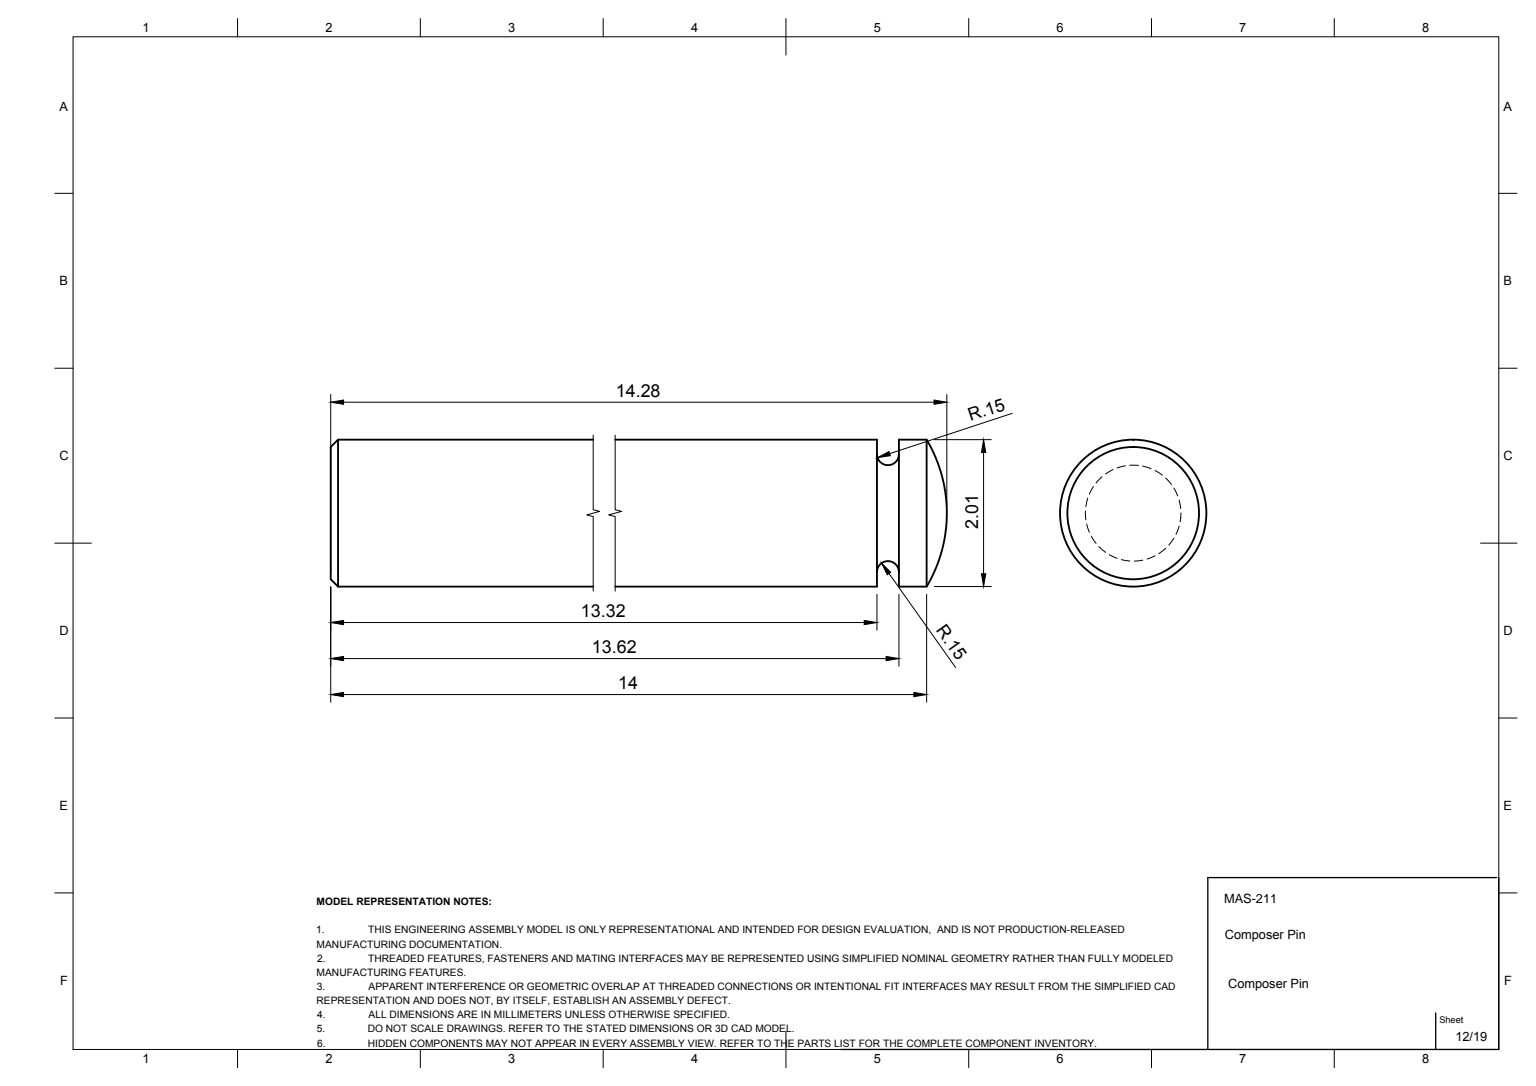
ISO-10303-21;
HEADER;
FILE_DESCRIPTION(
 (''),
 '2;1');
FILE_NAME ( 'Composer Pin.step', '2026-10-05T20:07:59+06:00', ( '' ), ( '' ), 'STEP AP214', 'Unspecified', '' );
FILE_SCHEMA (('AUTOMOTIVE_DESIGN { 1 0 10303 214 3 1 1 }'));
ENDSEC;
DATA;
#10=MECHANICAL_DESIGN_GEOMETRIC_PRESENTATION_REPRESENTATION('',(#329),#196741);
#17=(
BOUNDED_CURVE()
B_SPLINE_CURVE(2,(#114139,#114140,#114141,#114142,#114143,#114144,#114145,
#114146,#114147),.UNSPECIFIED.,.F.,.F.)
B_SPLINE_CURVE_WITH_KNOTS((3,2,2,2,3),(1.42918797785348,1.62618617063892,
1.86180561965816,2.09742506867739,2.29442326146283),.UNSPECIFIED.)
CURVE()
GEOMETRIC_REPRESENTATION_ITEM()
RATIONAL_B_SPLINE_CURVE((1.,1.,1.,0.707106781186548,1.,0.707106781186548,
1.,1.,1.))
REPRESENTATION_ITEM('')
) ;
#33=(
BOUNDED_SURFACE()
B_SPLINE_SURFACE(2,2,((#114004,#114005,#114006,#114007,#114008,#114009,
#114010,#114011,#114012),(#114013,#114014,#114015,#114016,#114017,#114018,
#114019,#114020,#114021),(#114022,#114023,#114024,#114025,#114026,#114027,
#114028,#114029,#114030)),.UNSPECIFIED.,.F.,.T.,.F.)
B_SPLINE_SURFACE_WITH_KNOTS((3,3),(3,2,2,2,3),(0.,1.05013832301181),(0.,
1.5707963267949,3.1415926535898,4.71238898038469,6.28318530717959),
 .UNSPECIFIED.)
GEOMETRIC_REPRESENTATION_ITEM()
RATIONAL_B_SPLINE_SURFACE(((1.,0.707106781186548,1.,0.707106781186548,1.,
0.707106781186548,1.,0.707106781186548,1.),(0.963886720506905,0.681570836366095,
0.963886720506905,0.681570836366095,0.963886720506905,0.681570836366095,
0.963886720506905,0.681570836366095,0.963886720506905),(1.,0.707106781186548,
1.,0.707106781186548,1.,0.707106781186548,1.,0.707106781186548,1.)))
REPRESENTATION_ITEM('')
SURFACE()
) ;
#34=(
BOUNDED_SURFACE()
B_SPLINE_SURFACE(2,1,((#114035,#114036),(#114037,#114038),(#114039,#114040),
(#114041,#114042),(#114043,#114044),(#114045,#114046),(#114047,#114048),
(#114049,#114050),(#114051,#114052)),.UNSPECIFIED.,.T.,.F.,.F.)
B_SPLINE_SURFACE_WITH_KNOTS((3,2,2,2,3),(2,2),(0.,1.5707963267949,3.1415926535898,
4.71238898038469,6.28318530717959),(0.,0.0454859585810009),
 .UNSPECIFIED.)
GEOMETRIC_REPRESENTATION_ITEM()
RATIONAL_B_SPLINE_SURFACE(((1.,1.),(0.707106781186548,0.707106781186548),
(1.,1.),(0.707106781186548,0.707106781186548),(1.,1.),(0.707106781186548,
0.707106781186548),(1.,1.),(0.707106781186548,0.707106781186548),(1.,1.)))
REPRESENTATION_ITEM('')
SURFACE()
) ;
#35=(
BOUNDED_SURFACE()
B_SPLINE_SURFACE(2,2,((#114056,#114057,#114058,#114059,#114060,#114061,
#114062,#114063,#114064),(#114065,#114066,#114067,#114068,#114069,#114070,
#114071,#114072,#114073),(#114074,#114075,#114076,#114077,#114078,#114079,
#114080,#114081,#114082),(#114083,#114084,#114085,#114086,#114087,#114088,
#114089,#114090,#114091),(#114092,#114093,#114094,#114095,#114096,#114097,
#114098,#114099,#114100),(#114101,#114102,#114103,#114104,#114105,#114106,
#114107,#114108,#114109),(#114110,#114111,#114112,#114113,#114114,#114115,
#114116,#114117,#114118),(#114119,#114120,#114121,#114122,#114123,#114124,
#114125,#114126,#114127),(#114128,#114129,#114130,#114131,#114132,#114133,
#114134,#114135,#114136)),.UNSPECIFIED.,.F.,.T.,.F.)
B_SPLINE_SURFACE_WITH_KNOTS((3,2,2,2,3),(3,2,2,2,3),(1.42918797785348,1.62618617063892,
1.86180561965816,2.09742506867739,2.29442326146283),(0.,1.5707963267949,
3.1415926535898,4.71238898038469,6.28318530717959),.UNSPECIFIED.)
GEOMETRIC_REPRESENTATION_ITEM()
RATIONAL_B_SPLINE_SURFACE(((1.,0.707106781186548,1.,0.707106781186548,1.,
0.707106781186548,1.,0.707106781186548,1.),(1.,0.707106781186548,1.,0.707106781186548,
1.,0.707106781186548,1.,0.707106781186548,1.),(1.,0.707106781186548,1.,
0.707106781186548,1.,0.707106781186548,1.,0.707106781186548,1.),(0.707106781186548,
0.5,0.707106781186548,0.5,0.707106781186548,0.5,0.707106781186548,0.5,0.707106781186548),
(1.,0.707106781186548,1.,0.707106781186548,1.,0.707106781186548,1.,0.707106781186548,
1.),(0.707106781186548,0.5,0.707106781186548,0.5,0.707106781186548,0.5,
0.707106781186548,0.5,0.707106781186548),(1.,0.707106781186548,1.,0.707106781186548,
1.,0.707106781186548,1.,0.707106781186548,1.),(1.,0.707106781186548,1.,
0.707106781186548,1.,0.707106781186548,1.,0.707106781186548,1.),(1.,0.707106781186548,
1.,0.707106781186548,1.,0.707106781186548,1.,0.707106781186548,1.)))
REPRESENTATION_ITEM('')
SURFACE()
) ;
#36=(
BOUNDED_SURFACE()
B_SPLINE_SURFACE(2,1,((#114148,#114149),(#114150,#114151),(#114152,#114153),
(#114154,#114155),(#114156,#114157),(#114158,#114159),(#114160,#114161),
(#114162,#114163),(#114164,#114165)),.UNSPECIFIED.,.T.,.F.,.F.)
B_SPLINE_SURFACE_WITH_KNOTS((3,2,2,2,3),(2,2),(0.,1.5707963267949,3.1415926535898,
4.71238898038469,6.28318530717959),(0.,1.586514041419),.UNSPECIFIED.)
GEOMETRIC_REPRESENTATION_ITEM()
RATIONAL_B_SPLINE_SURFACE(((1.,1.),(0.707106781186548,0.707106781186548),
(1.,1.),(0.707106781186548,0.707106781186548),(1.,1.),(0.707106781186548,
0.707106781186548),(1.,1.),(0.707106781186548,0.707106781186548),(1.,1.)))
REPRESENTATION_ITEM('')
SURFACE()
) ;
#37=(
BOUNDED_SURFACE()
B_SPLINE_SURFACE(1,2,((#114169,#114170,#114171,#114172,#114173,#114174,
#114175,#114176,#114177),(#114178,#114179,#114180,#114181,#114182,#114183,
#114184,#114185,#114186)),.UNSPECIFIED.,.F.,.T.,.F.)
B_SPLINE_SURFACE_WITH_KNOTS((2,2),(3,2,2,2,3),(15.5153736066212,15.6567949628585),
(0.,1.5707963267949,3.1415926535898,4.71238898038469,6.28318530717959),
 .UNSPECIFIED.)
GEOMETRIC_REPRESENTATION_ITEM()
RATIONAL_B_SPLINE_SURFACE(((1.,0.707106781186548,1.,0.707106781186548,1.,
0.707106781186548,1.,0.707106781186548,1.),(1.,0.707106781186548,1.,0.707106781186548,
1.,0.707106781186548,1.,0.707106781186548,1.)))
REPRESENTATION_ITEM('')
SURFACE()
) ;
#139=ELLIPSE('',#8975,0.90392506178254,0.899999999999994) ;
#140=ELLIPSE('',#8976,1.00436117975839,0.999999999999988) ;
#141=ELLIPSE('',#8978,1.00436117975839,0.999999999999988) ;
#142=ELLIPSE('',#8979,1.00436117975839,0.999999999999988) ;
#143=ELLIPSE('',#8980,1.00436117975839,0.999999999999998) ;
#329=STYLED_ITEM('',(#196765),#348) ;
#348=MANIFOLD_SOLID_BREP('Composer Pin',#8725) ;
#398=PLANE('',#8974) ;
#707=CIRCLE('',#8977,1.94783572104092) ;
#1030=FACE_OUTER_BOUND('',#1539,.T.) ;
#1031=FACE_OUTER_BOUND('',#1540,.T.) ;
#1032=FACE_OUTER_BOUND('',#1541,.T.) ;
#1033=FACE_OUTER_BOUND('',#1542,.T.) ;
#1034=FACE_OUTER_BOUND('',#1543,.T.) ;
#1035=FACE_OUTER_BOUND('',#1544,.T.) ;
#1539=EDGE_LOOP('',(#6448,#6449,#6450)) ;
#1540=EDGE_LOOP('',(#6451,#6452,#6453)) ;
#1541=EDGE_LOOP('',(#6454,#6455,#6456,#6457)) ;
#1542=EDGE_LOOP('',(#6458,#6459,#6460,#6461)) ;
#1543=EDGE_LOOP('',(#6462,#6463,#6464,#6465)) ;
#1544=EDGE_LOOP('',(#6466,#6467,#6468,#6469)) ;
#2034=LINE('',#114002,#2737) ;
#2035=LINE('',#114055,#2738) ;
#2036=LINE('',#114168,#2739) ;
#2037=LINE('',#114187,#2740) ;
#2737=VECTOR('',#10084,10.) ;
#2738=VECTOR('',#10093,10.) ;
#2739=VECTOR('',#10098,10.) ;
#2740=VECTOR('',#10099,10.) ;
#3736=VERTEX_POINT('',#114000) ;
#3737=VERTEX_POINT('',#114001) ;
#3738=VERTEX_POINT('',#114031) ;
#3739=VERTEX_POINT('',#114033) ;
#3740=VERTEX_POINT('',#114053) ;
#3741=VERTEX_POINT('',#114137) ;
#3742=VERTEX_POINT('',#114166) ;
#4732=EDGE_CURVE('',#3736,#3737,#2034,.T.) ;
#4733=EDGE_CURVE('',#3736,#3736,#139,.T.) ;
#4734=EDGE_CURVE('',#3738,#3738,#140,.T.) ;
#4735=EDGE_CURVE('',#3739,#3738,#707,.T.) ;
#4736=EDGE_CURVE('',#3740,#3740,#141,.T.) ;
#4737=EDGE_CURVE('',#3738,#3740,#2035,.T.) ;
#4738=EDGE_CURVE('',#3741,#3741,#142,.T.) ;
#4739=EDGE_CURVE('',#3740,#3741,#17,.T.) ;
#4740=EDGE_CURVE('',#3742,#3742,#143,.T.) ;
#4741=EDGE_CURVE('',#3741,#3742,#2036,.T.) ;
#4742=EDGE_CURVE('',#3742,#3736,#2037,.T.) ;
#6448=ORIENTED_EDGE('',*,*,#4732,.T.) ;
#6449=ORIENTED_EDGE('',*,*,#4732,.F.) ;
#6450=ORIENTED_EDGE('',*,*,#4733,.F.) ;
#6451=ORIENTED_EDGE('',*,*,#4734,.T.) ;
#6452=ORIENTED_EDGE('',*,*,#4735,.F.) ;
#6453=ORIENTED_EDGE('',*,*,#4735,.T.) ;
#6454=ORIENTED_EDGE('',*,*,#4736,.T.) ;
#6455=ORIENTED_EDGE('',*,*,#4737,.F.) ;
#6456=ORIENTED_EDGE('',*,*,#4734,.F.) ;
#6457=ORIENTED_EDGE('',*,*,#4737,.T.) ;
#6458=ORIENTED_EDGE('',*,*,#4738,.T.) ;
#6459=ORIENTED_EDGE('',*,*,#4739,.F.) ;
#6460=ORIENTED_EDGE('',*,*,#4736,.F.) ;
#6461=ORIENTED_EDGE('',*,*,#4739,.T.) ;
#6462=ORIENTED_EDGE('',*,*,#4740,.T.) ;
#6463=ORIENTED_EDGE('',*,*,#4741,.F.) ;
#6464=ORIENTED_EDGE('',*,*,#4738,.F.) ;
#6465=ORIENTED_EDGE('',*,*,#4741,.T.) ;
#6466=ORIENTED_EDGE('',*,*,#4733,.T.) ;
#6467=ORIENTED_EDGE('',*,*,#4742,.F.) ;
#6468=ORIENTED_EDGE('',*,*,#4740,.F.) ;
#6469=ORIENTED_EDGE('',*,*,#4742,.T.) ;
#8413=ADVANCED_FACE('',(#1030),#398,.T.) ;
#8414=ADVANCED_FACE('',(#1031),#33,.T.) ;
#8415=ADVANCED_FACE('',(#1032),#34,.F.) ;
#8416=ADVANCED_FACE('',(#1033),#35,.T.) ;
#8417=ADVANCED_FACE('',(#1034),#36,.F.) ;
#8418=ADVANCED_FACE('',(#1035),#37,.T.) ;
#8725=CLOSED_SHELL('',(#8413,#8414,#8415,#8416,#8417,#8418)) ;
#8974=AXIS2_PLACEMENT_3D('',#113999,#10082,#10083) ;
#8975=AXIS2_PLACEMENT_3D('',#114003,#10085,#10086) ;
#8976=AXIS2_PLACEMENT_3D('',#114032,#10087,#10088) ;
#8977=AXIS2_PLACEMENT_3D('',#114034,#10089,#10090) ;
#8978=AXIS2_PLACEMENT_3D('',#114054,#10091,#10092) ;
#8979=AXIS2_PLACEMENT_3D('',#114138,#10094,#10095) ;
#8980=AXIS2_PLACEMENT_3D('',#114167,#10096,#10097) ;
#10082=DIRECTION('center_axis',(-4.35747896024226E-15,-1.,5.94017881872706E-16)) ;
#10083=DIRECTION('ref_axis',(0.,-5.94017881872706E-16,-1.)) ;
#10084=DIRECTION('',(0.323867587736079,-1.97204328484321E-15,-0.946102418141933)) ;
#10085=DIRECTION('center_axis',(0.,1.,0.)) ;
#10086=DIRECTION('ref_axis',(0.946102418142542,0.,0.3238675877343)) ;
#10087=DIRECTION('center_axis',(1.67995222306785E-15,1.,-3.91636034436018E-16)) ;
#10088=DIRECTION('ref_axis',(0.946102418142689,-1.46256864286623E-15,0.323867587733871)) ;
#10089=DIRECTION('center_axis',(0.946102418141937,-3.68441630821444E-14,
0.323867587736069)) ;
#10090=DIRECTION('ref_axis',(-0.166270483818289,0.858155219939116,0.485719821195387)) ;
#10091=DIRECTION('center_axis',(1.78081198063816E-15,1.,9.26117405585395E-16)) ;
#10092=DIRECTION('ref_axis',(0.946102418142689,-1.98476993124453E-15,0.323867587733871)) ;
#10093=DIRECTION('',(-2.3431716883402E-14,-1.,4.6863433766804E-14)) ;
#10094=DIRECTION('center_axis',(1.67995222306785E-15,1.,-3.91636034436018E-16)) ;
#10095=DIRECTION('ref_axis',(0.946102418142689,-1.46256864286623E-15,0.323867587733871)) ;
#10096=DIRECTION('center_axis',(0.,1.,0.)) ;
#10097=DIRECTION('ref_axis',(0.94610241814253,0.,0.323867587734335)) ;
#10098=DIRECTION('',(-6.71796199601783E-16,-1.,1.34359239920357E-15)) ;
#10099=DIRECTION('',(0.229008967494671,-0.707106781186611,-0.668995435565098)) ;
#113999=CARTESIAN_POINT('Origin',(-34.1140302566115,0.00967047744422178,
126.985310472154)) ;
#114000=CARTESIAN_POINT('',(-34.2597706710927,0.00967047744422267,127.411056560318)) ;
#114001=CARTESIAN_POINT('',(-33.9682898421302,0.00967047744422267,126.55956438399)) ;
#114002=CARTESIAN_POINT('',(-34.2597706710927,0.00967047744422267,127.411056560318)) ;
#114003=CARTESIAN_POINT('Origin',(-33.9682898421302,0.00967047744422267,
126.55956438399)) ;
#114004=CARTESIAN_POINT('Ctrl Pts',(-33.9682898421302,14.28596080689,126.55956438399)) ;
#114005=CARTESIAN_POINT('Ctrl Pts',(-33.9682898421302,14.28596080689,126.55956438399)) ;
#114006=CARTESIAN_POINT('Ctrl Pts',(-33.9682898421302,14.28596080689,126.55956438399)) ;
#114007=CARTESIAN_POINT('Ctrl Pts',(-33.9682898421302,14.28596080689,126.55956438399)) ;
#114008=CARTESIAN_POINT('Ctrl Pts',(-33.9682898421302,14.28596080689,126.55956438399)) ;
#114009=CARTESIAN_POINT('Ctrl Pts',(-33.9682898421302,14.28596080689,126.55956438399)) ;
#114010=CARTESIAN_POINT('Ctrl Pts',(-33.9682898421302,14.28596080689,126.55956438399)) ;
#114011=CARTESIAN_POINT('Ctrl Pts',(-33.9682898421302,14.28596080689,126.55956438399)) ;
#114012=CARTESIAN_POINT('Ctrl Pts',(-33.9682898421302,14.28596080689,126.55956438399)) ;
#114013=CARTESIAN_POINT('Ctrl Pts',(-34.1425850701396,14.28596080689,127.068726593901)) ;
#114014=CARTESIAN_POINT('Ctrl Pts',(-33.631202312305,14.28596080689,127.243781954731)) ;
#114015=CARTESIAN_POINT('Ctrl Pts',(-33.4569070842956,14.28596080689,126.73461974482)) ;
#114016=CARTESIAN_POINT('Ctrl Pts',(-33.2826118562863,14.28596080689,126.225457534909)) ;
#114017=CARTESIAN_POINT('Ctrl Pts',(-33.7939946141209,14.28596080689,126.050402174079)) ;
#114018=CARTESIAN_POINT('Ctrl Pts',(-34.3053773719555,14.28596080689,125.875346813249)) ;
#114019=CARTESIAN_POINT('Ctrl Pts',(-34.4796725999648,14.28596080689,126.38450902316)) ;
#114020=CARTESIAN_POINT('Ctrl Pts',(-34.6539678279742,14.28596080689,126.893671233071)) ;
#114021=CARTESIAN_POINT('Ctrl Pts',(-34.1425850701396,14.28596080689,127.068726593901)) ;
#114022=CARTESIAN_POINT('Ctrl Pts',(-34.2921574298663,14.0096704774442,
127.505666802132)) ;
#114023=CARTESIAN_POINT('Ctrl Pts',(-33.341928889009,14.0096704774442,127.830946834636)) ;
#114024=CARTESIAN_POINT('Ctrl Pts',(-33.018061301273,14.0096704774442,126.884844416494)) ;
#114025=CARTESIAN_POINT('Ctrl Pts',(-32.6941937135369,14.0096704774442,
125.938741998352)) ;
#114026=CARTESIAN_POINT('Ctrl Pts',(-33.6444222543942,14.0096704774442,
125.613461965848)) ;
#114027=CARTESIAN_POINT('Ctrl Pts',(-34.5946507952514,14.0096704774442,
125.288181933344)) ;
#114028=CARTESIAN_POINT('Ctrl Pts',(-34.9185183829875,14.0096704774442,
126.234284351486)) ;
#114029=CARTESIAN_POINT('Ctrl Pts',(-35.2423859707236,14.0096704774442,
127.180386769628)) ;
#114030=CARTESIAN_POINT('Ctrl Pts',(-34.2921574298663,14.0096704774442,
127.505666802132)) ;
#114031=CARTESIAN_POINT('',(-34.2921574298663,14.0096704774442,127.505666802132)) ;
#114032=CARTESIAN_POINT('Origin',(-33.9682898421302,14.0096704774442,126.55956438399)) ;
#114033=CARTESIAN_POINT('',(-33.9682898421302,14.28596080689,126.55956438399)) ;
#114034=CARTESIAN_POINT('Origin',(-33.9682898421303,12.3381250858491,126.55956438399)) ;
#114035=CARTESIAN_POINT('Ctrl Pts',(-34.2921574298663,14.0096704774442,
127.505666802132)) ;
#114036=CARTESIAN_POINT('Ctrl Pts',(-34.2921574298663,13.5548108916342,
127.505666802132)) ;
#114037=CARTESIAN_POINT('Ctrl Pts',(-33.341928889009,14.0096704774442,127.830946834636)) ;
#114038=CARTESIAN_POINT('Ctrl Pts',(-33.341928889009,13.5548108916342,127.830946834636)) ;
#114039=CARTESIAN_POINT('Ctrl Pts',(-33.018061301273,14.0096704774442,126.884844416494)) ;
#114040=CARTESIAN_POINT('Ctrl Pts',(-33.018061301273,13.5548108916342,126.884844416494)) ;
#114041=CARTESIAN_POINT('Ctrl Pts',(-32.6941937135369,14.0096704774442,
125.938741998352)) ;
#114042=CARTESIAN_POINT('Ctrl Pts',(-32.6941937135369,13.5548108916342,
125.938741998352)) ;
#114043=CARTESIAN_POINT('Ctrl Pts',(-33.6444222543942,14.0096704774442,
125.613461965848)) ;
#114044=CARTESIAN_POINT('Ctrl Pts',(-33.6444222543942,13.5548108916342,
125.613461965848)) ;
#114045=CARTESIAN_POINT('Ctrl Pts',(-34.5946507952514,14.0096704774442,
125.288181933344)) ;
#114046=CARTESIAN_POINT('Ctrl Pts',(-34.5946507952514,13.5548108916342,
125.288181933344)) ;
#114047=CARTESIAN_POINT('Ctrl Pts',(-34.9185183829875,14.0096704774442,
126.234284351486)) ;
#114048=CARTESIAN_POINT('Ctrl Pts',(-34.9185183829875,13.5548108916342,
126.234284351486)) ;
#114049=CARTESIAN_POINT('Ctrl Pts',(-35.2423859707236,14.0096704774442,
127.180386769628)) ;
#114050=CARTESIAN_POINT('Ctrl Pts',(-35.2423859707236,13.5548108916342,
127.180386769628)) ;
#114051=CARTESIAN_POINT('Ctrl Pts',(-34.2921574298663,14.0096704774442,
127.505666802132)) ;
#114052=CARTESIAN_POINT('Ctrl Pts',(-34.2921574298663,13.5548108916342,
127.505666802132)) ;
#114053=CARTESIAN_POINT('',(-34.2921574298663,13.6306208226026,127.505666802132)) ;
#114054=CARTESIAN_POINT('Origin',(-33.9682898421302,13.6306208226026,126.55956438399)) ;
#114055=CARTESIAN_POINT('',(-34.2921574298663,14.0096704774442,127.505666802132)) ;
#114056=CARTESIAN_POINT('Ctrl Pts',(-34.2921574298663,13.6306208226026,
127.505666802132)) ;
#114057=CARTESIAN_POINT('Ctrl Pts',(-33.341928889009,13.6306208226025,127.830946834636)) ;
#114058=CARTESIAN_POINT('Ctrl Pts',(-33.018061301273,13.6306208226026,126.884844416494)) ;
#114059=CARTESIAN_POINT('Ctrl Pts',(-32.6941937135369,13.6306208226025,
125.938741998352)) ;
#114060=CARTESIAN_POINT('Ctrl Pts',(-33.6444222543942,13.6306208226026,
125.613461965848)) ;
#114061=CARTESIAN_POINT('Ctrl Pts',(-34.5946507952514,13.6306208226025,
125.288181933344)) ;
#114062=CARTESIAN_POINT('Ctrl Pts',(-34.9185183829875,13.6306208226026,
126.234284351486)) ;
#114063=CARTESIAN_POINT('Ctrl Pts',(-35.2423859707236,13.6306208226025,
127.180386769628)) ;
#114064=CARTESIAN_POINT('Ctrl Pts',(-34.2921574298663,13.6306208226026,
127.505666802132)) ;
#114065=CARTESIAN_POINT('Ctrl Pts',(-34.2602567651234,13.6306208226026,
127.41247656885)) ;
#114066=CARTESIAN_POINT('Ctrl Pts',(-33.4036248769071,13.6306208226025,
127.705716812078)) ;
#114067=CARTESIAN_POINT('Ctrl Pts',(-33.111657953914,13.6306208226026,126.852804627218)) ;
#114068=CARTESIAN_POINT('Ctrl Pts',(-32.8196910309208,13.6306208226025,
125.999892442358)) ;
#114069=CARTESIAN_POINT('Ctrl Pts',(-33.676322919137,13.6306208226026,125.70665219913)) ;
#114070=CARTESIAN_POINT('Ctrl Pts',(-34.5329548073533,13.6306208226025,
125.413411955902)) ;
#114071=CARTESIAN_POINT('Ctrl Pts',(-34.8249217303465,13.6306208226026,
126.266324140762)) ;
#114072=CARTESIAN_POINT('Ctrl Pts',(-35.1168886533397,13.6306208226025,
127.119236325622)) ;
#114073=CARTESIAN_POINT('Ctrl Pts',(-34.2602567651234,13.6306208226026,
127.41247656885)) ;
#114074=CARTESIAN_POINT('Ctrl Pts',(-34.2283561003805,13.6306208226026,
127.319286335568)) ;
#114075=CARTESIAN_POINT('Ctrl Pts',(-33.4653208648053,13.6306208226025,
127.580486789519)) ;
#114076=CARTESIAN_POINT('Ctrl Pts',(-33.205254606555,13.6306208226026,126.820764837941)) ;
#114077=CARTESIAN_POINT('Ctrl Pts',(-32.9451883483047,13.6306208226025,
126.061042886363)) ;
#114078=CARTESIAN_POINT('Ctrl Pts',(-33.70822358388,13.6306208226026,125.799842432412)) ;
#114079=CARTESIAN_POINT('Ctrl Pts',(-34.4712588194552,13.6306208226025,
125.53864197846)) ;
#114080=CARTESIAN_POINT('Ctrl Pts',(-34.7313250777055,13.6306208226026,
126.298363930038)) ;
#114081=CARTESIAN_POINT('Ctrl Pts',(-34.9913913359558,13.6306208226025,
127.058085881616)) ;
#114082=CARTESIAN_POINT('Ctrl Pts',(-34.2283561003805,13.6306208226026,
127.319286335568)) ;
#114083=CARTESIAN_POINT('Ctrl Pts',(-34.1797759622201,13.6306208226025,
127.177370972847)) ;
#114084=CARTESIAN_POINT('Ctrl Pts',(-33.5592750077734,13.6306208226025,
127.389779421923)) ;
#114085=CARTESIAN_POINT('Ctrl Pts',(-33.3477888876835,13.6306208226025,
126.771972833066)) ;
#114086=CARTESIAN_POINT('Ctrl Pts',(-33.1363027675937,13.6306208226025,
126.154166244209)) ;
#114087=CARTESIAN_POINT('Ctrl Pts',(-33.7568037220404,13.6306208226025,
125.941757795133)) ;
#114088=CARTESIAN_POINT('Ctrl Pts',(-34.377304676487,13.6306208226025,125.729349346057)) ;
#114089=CARTESIAN_POINT('Ctrl Pts',(-34.5887907965769,13.6306208226025,
126.347155934914)) ;
#114090=CARTESIAN_POINT('Ctrl Pts',(-34.8002769166668,13.6306208226025,
126.964962523771)) ;
#114091=CARTESIAN_POINT('Ctrl Pts',(-34.1797759622201,13.6306208226025,
127.177370972847)) ;
#114092=CARTESIAN_POINT('Ctrl Pts',(-34.1797759622201,13.4806208226026,
127.177370972847)) ;
#114093=CARTESIAN_POINT('Ctrl Pts',(-33.5592750077734,13.4806208226026,
127.389779421923)) ;
#114094=CARTESIAN_POINT('Ctrl Pts',(-33.3477888876836,13.4806208226026,
126.771972833066)) ;
#114095=CARTESIAN_POINT('Ctrl Pts',(-33.1363027675937,13.4806208226026,
126.154166244209)) ;
#114096=CARTESIAN_POINT('Ctrl Pts',(-33.7568037220404,13.4806208226026,
125.941757795133)) ;
#114097=CARTESIAN_POINT('Ctrl Pts',(-34.377304676487,13.4806208226026,125.729349346057)) ;
#114098=CARTESIAN_POINT('Ctrl Pts',(-34.5887907965769,13.4806208226026,
126.347155934914)) ;
#114099=CARTESIAN_POINT('Ctrl Pts',(-34.8002769166668,13.4806208226026,
126.964962523771)) ;
#114100=CARTESIAN_POINT('Ctrl Pts',(-34.1797759622201,13.4806208226026,
127.177370972847)) ;
#114101=CARTESIAN_POINT('Ctrl Pts',(-34.1797759622201,13.3306208226026,
127.177370972847)) ;
#114102=CARTESIAN_POINT('Ctrl Pts',(-33.5592750077734,13.3306208226026,
127.389779421923)) ;
#114103=CARTESIAN_POINT('Ctrl Pts',(-33.3477888876835,13.3306208226026,
126.771972833066)) ;
#114104=CARTESIAN_POINT('Ctrl Pts',(-33.1363027675937,13.3306208226026,
126.154166244209)) ;
#114105=CARTESIAN_POINT('Ctrl Pts',(-33.7568037220404,13.3306208226026,
125.941757795133)) ;
#114106=CARTESIAN_POINT('Ctrl Pts',(-34.377304676487,13.3306208226026,125.729349346057)) ;
#114107=CARTESIAN_POINT('Ctrl Pts',(-34.5887907965769,13.3306208226026,
126.347155934914)) ;
#114108=CARTESIAN_POINT('Ctrl Pts',(-34.8002769166668,13.3306208226026,
126.964962523771)) ;
#114109=CARTESIAN_POINT('Ctrl Pts',(-34.1797759622201,13.3306208226026,
127.177370972847)) ;
#114110=CARTESIAN_POINT('Ctrl Pts',(-34.2283561003805,13.3306208226026,
127.319286335568)) ;
#114111=CARTESIAN_POINT('Ctrl Pts',(-33.4653208648053,13.3306208226026,
127.580486789519)) ;
#114112=CARTESIAN_POINT('Ctrl Pts',(-33.205254606555,13.3306208226026,126.820764837941)) ;
#114113=CARTESIAN_POINT('Ctrl Pts',(-32.9451883483047,13.3306208226026,
126.061042886363)) ;
#114114=CARTESIAN_POINT('Ctrl Pts',(-33.70822358388,13.3306208226026,125.799842432412)) ;
#114115=CARTESIAN_POINT('Ctrl Pts',(-34.4712588194552,13.3306208226026,
125.53864197846)) ;
#114116=CARTESIAN_POINT('Ctrl Pts',(-34.7313250777055,13.3306208226026,
126.298363930038)) ;
#114117=CARTESIAN_POINT('Ctrl Pts',(-34.9913913359558,13.3306208226026,
127.058085881616)) ;
#114118=CARTESIAN_POINT('Ctrl Pts',(-34.2283561003805,13.3306208226026,
127.319286335568)) ;
#114119=CARTESIAN_POINT('Ctrl Pts',(-34.2602567651234,13.3306208226026,
127.41247656885)) ;
#114120=CARTESIAN_POINT('Ctrl Pts',(-33.4036248769071,13.3306208226026,
127.705716812078)) ;
#114121=CARTESIAN_POINT('Ctrl Pts',(-33.111657953914,13.3306208226026,126.852804627218)) ;
#114122=CARTESIAN_POINT('Ctrl Pts',(-32.8196910309208,13.3306208226026,
125.999892442358)) ;
#114123=CARTESIAN_POINT('Ctrl Pts',(-33.676322919137,13.3306208226026,125.70665219913)) ;
#114124=CARTESIAN_POINT('Ctrl Pts',(-34.5329548073533,13.3306208226026,
125.413411955902)) ;
#114125=CARTESIAN_POINT('Ctrl Pts',(-34.8249217303465,13.3306208226026,
126.266324140762)) ;
#114126=CARTESIAN_POINT('Ctrl Pts',(-35.1168886533397,13.3306208226026,
127.119236325622)) ;
#114127=CARTESIAN_POINT('Ctrl Pts',(-34.2602567651234,13.3306208226026,
127.41247656885)) ;
#114128=CARTESIAN_POINT('Ctrl Pts',(-34.2921574298663,13.3306208226026,
127.505666802132)) ;
#114129=CARTESIAN_POINT('Ctrl Pts',(-33.341928889009,13.3306208226026,127.830946834636)) ;
#114130=CARTESIAN_POINT('Ctrl Pts',(-33.018061301273,13.3306208226026,126.884844416494)) ;
#114131=CARTESIAN_POINT('Ctrl Pts',(-32.6941937135369,13.3306208226026,
125.938741998352)) ;
#114132=CARTESIAN_POINT('Ctrl Pts',(-33.6444222543942,13.3306208226026,
125.613461965848)) ;
#114133=CARTESIAN_POINT('Ctrl Pts',(-34.5946507952514,13.3306208226026,
125.288181933344)) ;
#114134=CARTESIAN_POINT('Ctrl Pts',(-34.9185183829875,13.3306208226026,
126.234284351486)) ;
#114135=CARTESIAN_POINT('Ctrl Pts',(-35.2423859707236,13.3306208226026,
127.180386769628)) ;
#114136=CARTESIAN_POINT('Ctrl Pts',(-34.2921574298663,13.3306208226026,
127.505666802132)) ;
#114137=CARTESIAN_POINT('',(-34.2921574298663,13.3306208226026,127.505666802132)) ;
#114138=CARTESIAN_POINT('Origin',(-33.9682898421302,13.3306208226026,126.55956438399)) ;
#114139=CARTESIAN_POINT('Ctrl Pts',(-34.2921574298663,13.6306208226026,
127.505666802132)) ;
#114140=CARTESIAN_POINT('Ctrl Pts',(-34.2602567651234,13.6306208226026,
127.41247656885)) ;
#114141=CARTESIAN_POINT('Ctrl Pts',(-34.2283561003805,13.6306208226026,
127.319286335568)) ;
#114142=CARTESIAN_POINT('Ctrl Pts',(-34.1797759622201,13.6306208226025,
127.177370972847)) ;
#114143=CARTESIAN_POINT('Ctrl Pts',(-34.1797759622201,13.4806208226026,
127.177370972847)) ;
#114144=CARTESIAN_POINT('Ctrl Pts',(-34.1797759622201,13.3306208226026,
127.177370972847)) ;
#114145=CARTESIAN_POINT('Ctrl Pts',(-34.2283561003805,13.3306208226026,
127.319286335568)) ;
#114146=CARTESIAN_POINT('Ctrl Pts',(-34.2602567651234,13.3306208226026,
127.41247656885)) ;
#114147=CARTESIAN_POINT('Ctrl Pts',(-34.2921574298663,13.3306208226026,
127.505666802132)) ;
#114148=CARTESIAN_POINT('Ctrl Pts',(-34.2921574298663,13.3306208226026,
127.505666802132)) ;
#114149=CARTESIAN_POINT('Ctrl Pts',(-34.2921574298663,-2.53451959158744,
127.505666802132)) ;
#114150=CARTESIAN_POINT('Ctrl Pts',(-33.341928889009,13.3306208226026,127.830946834636)) ;
#114151=CARTESIAN_POINT('Ctrl Pts',(-33.341928889009,-2.53451959158744,
127.830946834636)) ;
#114152=CARTESIAN_POINT('Ctrl Pts',(-33.018061301273,13.3306208226026,126.884844416494)) ;
#114153=CARTESIAN_POINT('Ctrl Pts',(-33.018061301273,-2.53451959158744,
126.884844416494)) ;
#114154=CARTESIAN_POINT('Ctrl Pts',(-32.6941937135369,13.3306208226026,
125.938741998352)) ;
#114155=CARTESIAN_POINT('Ctrl Pts',(-32.6941937135369,-2.53451959158744,
125.938741998352)) ;
#114156=CARTESIAN_POINT('Ctrl Pts',(-33.6444222543942,13.3306208226026,
125.613461965848)) ;
#114157=CARTESIAN_POINT('Ctrl Pts',(-33.6444222543942,-2.53451959158744,
125.613461965848)) ;
#114158=CARTESIAN_POINT('Ctrl Pts',(-34.5946507952514,13.3306208226026,
125.288181933344)) ;
#114159=CARTESIAN_POINT('Ctrl Pts',(-34.5946507952514,-2.53451959158744,
125.288181933344)) ;
#114160=CARTESIAN_POINT('Ctrl Pts',(-34.9185183829875,13.3306208226026,
126.234284351486)) ;
#114161=CARTESIAN_POINT('Ctrl Pts',(-34.9185183829875,-2.53451959158744,
126.234284351486)) ;
#114162=CARTESIAN_POINT('Ctrl Pts',(-35.2423859707236,13.3306208226026,
127.180386769628)) ;
#114163=CARTESIAN_POINT('Ctrl Pts',(-35.2423859707236,-2.53451959158744,
127.180386769628)) ;
#114164=CARTESIAN_POINT('Ctrl Pts',(-34.2921574298663,13.3306208226026,
127.505666802132)) ;
#114165=CARTESIAN_POINT('Ctrl Pts',(-34.2921574298663,-2.53451959158744,
127.505666802132)) ;
#114166=CARTESIAN_POINT('',(-34.2921574298663,0.109670477444222,127.505666802132)) ;
#114167=CARTESIAN_POINT('Origin',(-33.9682898421302,0.109670477444222,126.55956438399)) ;
#114168=CARTESIAN_POINT('',(-34.2921574298663,13.3306208226026,127.505666802132)) ;
#114169=CARTESIAN_POINT('Ctrl Pts',(-34.2921574298663,0.109670477444222,
127.505666802132)) ;
#114170=CARTESIAN_POINT('Ctrl Pts',(-33.341928889009,0.109670477444222,
127.830946834636)) ;
#114171=CARTESIAN_POINT('Ctrl Pts',(-33.018061301273,0.109670477444222,
126.884844416494)) ;
#114172=CARTESIAN_POINT('Ctrl Pts',(-32.6941937135369,0.109670477444222,
125.938741998352)) ;
#114173=CARTESIAN_POINT('Ctrl Pts',(-33.6444222543942,0.109670477444222,
125.613461965848)) ;
#114174=CARTESIAN_POINT('Ctrl Pts',(-34.5946507952514,0.109670477444222,
125.288181933344)) ;
#114175=CARTESIAN_POINT('Ctrl Pts',(-34.9185183829875,0.109670477444222,
126.234284351486)) ;
#114176=CARTESIAN_POINT('Ctrl Pts',(-35.2423859707236,0.109670477444222,
127.180386769628)) ;
#114177=CARTESIAN_POINT('Ctrl Pts',(-34.2921574298663,0.109670477444222,
127.505666802132)) ;
#114178=CARTESIAN_POINT('Ctrl Pts',(-34.2597706710927,0.00967047744422267,
127.411056560318)) ;
#114179=CARTESIAN_POINT('Ctrl Pts',(-33.4045649843211,0.00967047744422267,
127.703808589571)) ;
#114180=CARTESIAN_POINT('Ctrl Pts',(-33.1130841553587,0.00967047744422267,
126.852316413244)) ;
#114181=CARTESIAN_POINT('Ctrl Pts',(-32.8216033263962,0.00967047744422267,
126.000824236916)) ;
#114182=CARTESIAN_POINT('Ctrl Pts',(-33.6768090131678,0.00967047744422267,
125.708072207662)) ;
#114183=CARTESIAN_POINT('Ctrl Pts',(-34.5320146999393,0.00967047744422267,
125.415320178408)) ;
#114184=CARTESIAN_POINT('Ctrl Pts',(-34.8234955289018,0.00967047744422267,
126.266812354736)) ;
#114185=CARTESIAN_POINT('Ctrl Pts',(-35.1149763578642,0.00967047744422267,
127.118304531064)) ;
#114186=CARTESIAN_POINT('Ctrl Pts',(-34.2597706710927,0.00967047744422267,
127.411056560318)) ;
#114187=CARTESIAN_POINT('',(-34.2921574298663,0.109670477444222,127.505666802132)) ;
#196737=UNCERTAINTY_MEASURE_WITH_UNIT(LENGTH_MEASURE(0.01),#196742,
'DISTANCE_ACCURACY_VALUE',
'Maximum model space distance between geometric entities at asserted c
onnectivities') ;
#196738=UNCERTAINTY_MEASURE_WITH_UNIT(LENGTH_MEASURE(0.01),#196742,
'DISTANCE_ACCURACY_VALUE',
'Maximum model space distance between geometric entities at asserted c
onnectivities') ;
#196740=(
GEOMETRIC_REPRESENTATION_CONTEXT(3)
GLOBAL_UNCERTAINTY_ASSIGNED_CONTEXT((#196737))
GLOBAL_UNIT_ASSIGNED_CONTEXT((#196742,#196744,#196745))
REPRESENTATION_CONTEXT('','3D')
) ;
#196741=(
GEOMETRIC_REPRESENTATION_CONTEXT(3)
GLOBAL_UNCERTAINTY_ASSIGNED_CONTEXT((#196738))
GLOBAL_UNIT_ASSIGNED_CONTEXT((#196742,#196744,#196745))
REPRESENTATION_CONTEXT('','3D')
) ;
#196742=(
LENGTH_UNIT()
NAMED_UNIT(*)
SI_UNIT(.MILLI.,.METRE.)
) ;
#196744=(
NAMED_UNIT(*)
PLANE_ANGLE_UNIT()
SI_UNIT($,.RADIAN.)
) ;
#196745=(
NAMED_UNIT(*)
SI_UNIT($,.STERADIAN.)
SOLID_ANGLE_UNIT()
) ;
#196753=PRODUCT_DEFINITION_CONTEXT('part definition',#196761,'design') ;
#196761=APPLICATION_CONTEXT(
'Core Data for Automotive Mechanical Design Process') ;
#196762=PRODUCT_CONTEXT('part definition',#196761,'mechanical') ;
#196765=PRESENTATION_STYLE_ASSIGNMENT((#196767)) ;
#196767=SURFACE_STYLE_USAGE(.BOTH.,#196769) ;
#196769=SURFACE_SIDE_STYLE('',(#196771)) ;
#196771=SURFACE_STYLE_FILL_AREA(#196773) ;
#196773=FILL_AREA_STYLE('Steel - Satin',(#196775)) ;
#196775=FILL_AREA_STYLE_COLOUR('Steel - Satin',#196777) ;
#196777=COLOUR_RGB('Steel - Satin', 0.09019608, 0.27058824, 0.51372549) ;
#197019=CARTESIAN_POINT ( '', ( 0.0, 0.0, 0.0 ) ) ;
#197020=DIRECTION ( '', ( 0.0, 0.0, 1.0 ) ) ;
#197021=DIRECTION ( '', ( 1.0, 0.0, 0.0 ) ) ;
#197022=AXIS2_PLACEMENT_3D ( '', #197019, #197020, #197021 ) ;
#197023=ADVANCED_BREP_SHAPE_REPRESENTATION ( 'Composer Pin', ( #348, #197022, #197033, #197368, #197498 ), #196740 ) ;
#197024=PRODUCT( 'Composer Pin', 'Composer Pin', '', ( #196762 ) ) ;
#197025=PRODUCT_DEFINITION_FORMATION ( '', '', #197024 ) ;
#197026=PRODUCT_DEFINITION( 'Composer Pin', 'Composer Pin', #197025, #196753 ) ;
#197027=PRODUCT_DEFINITION_SHAPE ( '', '', #197026 ) ;
#197028=SHAPE_DEFINITION_REPRESENTATION ( #197027, #197023 ) ;
#197030=CARTESIAN_POINT ( '', ( 0.0, 0.0, 0.0 ) ) ;
#197031=DIRECTION ( '', ( 0.0, 0.0, 1.0 ) ) ;
#197032=DIRECTION ( '', ( 1.0, 0.0, 0.0 ) ) ;
#197033=AXIS2_PLACEMENT_3D ( '', #197030, #197031, #197032 ) ;
#197365=CARTESIAN_POINT ( '', ( 0.0, 0.0, 0.0 ) ) ;
#197366=DIRECTION ( '', ( 0.0, 0.0, 1.0 ) ) ;
#197367=DIRECTION ( '', ( 1.0, 0.0, 0.0 ) ) ;
#197368=AXIS2_PLACEMENT_3D ( '', #197365, #197366, #197367 ) ;
#197495=CARTESIAN_POINT ( '', ( 0.0, 0.0, 0.0 ) ) ;
#197496=DIRECTION ( '', ( 0.0, 0.0, 1.0 ) ) ;
#197497=DIRECTION ( '', ( 1.0, 0.0, 0.0 ) ) ;
#197498=AXIS2_PLACEMENT_3D ( '', #197495, #197496, #197497 ) ;
ENDSEC;
END-ISO-10303-21;
